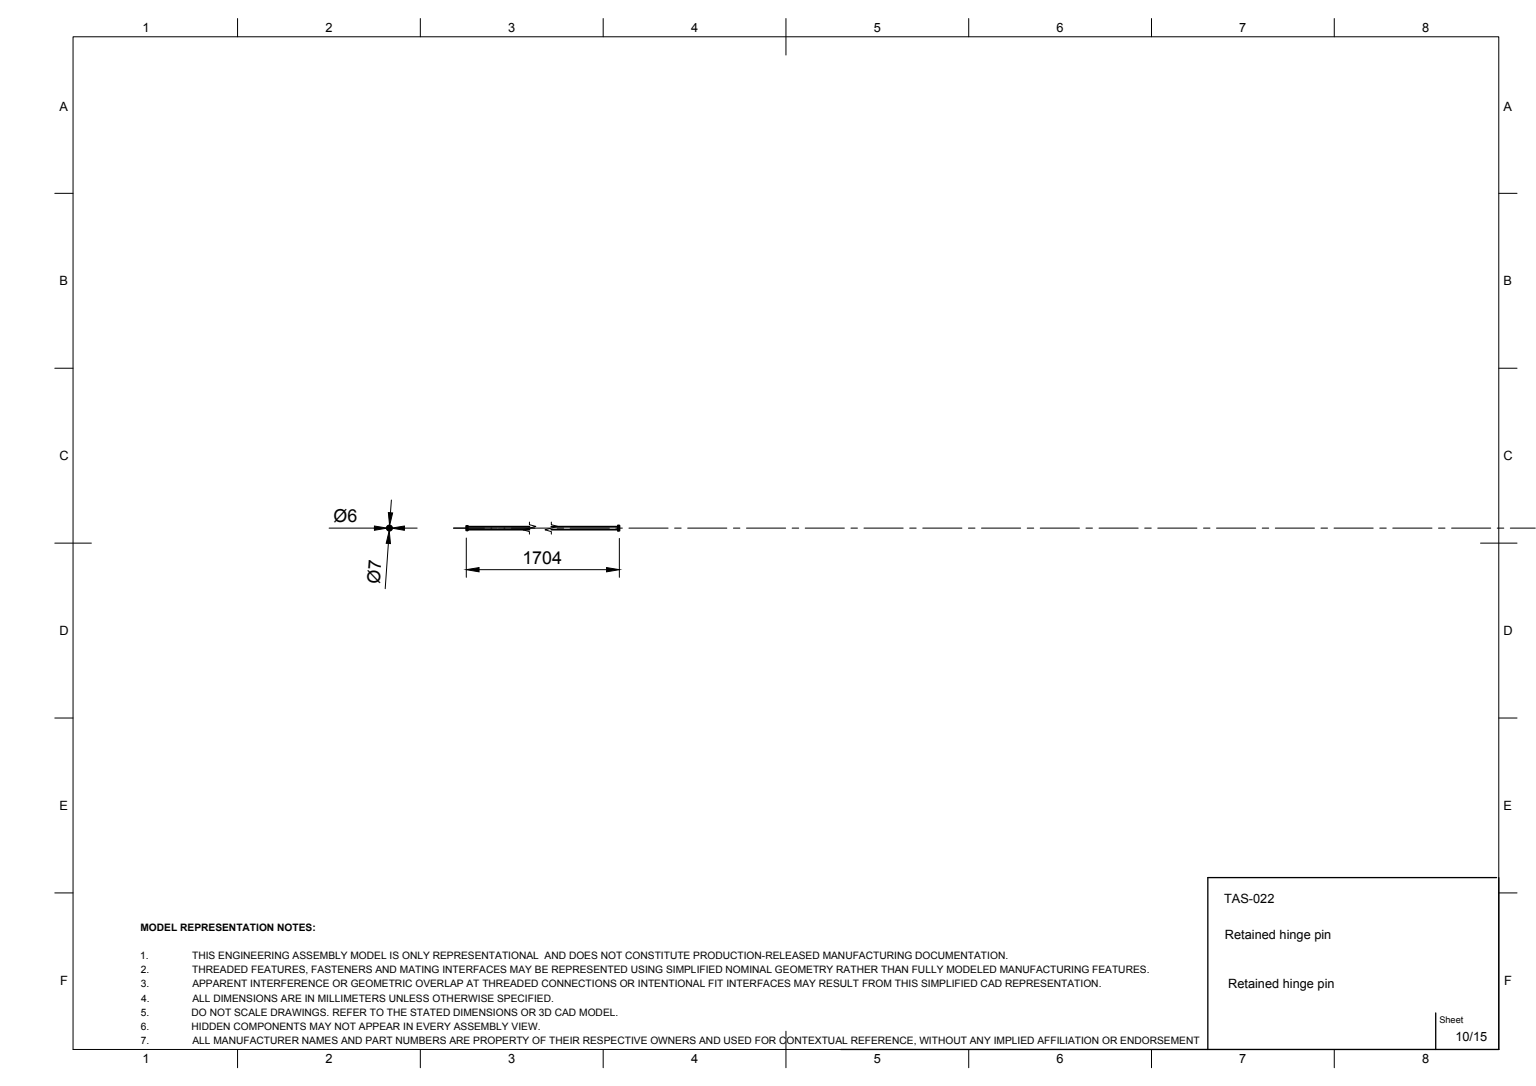
ISO-10303-21;
HEADER;
/* Generated by software containing ST-Developer
 * from STEP Tools, Inc. (www.steptools.com) 
 */

FILE_DESCRIPTION(
/* description */ (''),
/* implementation_level */ '2;1');

FILE_NAME(
/* name */ 'Retained hinge pin.step',
/* time_stamp */ '2026-11-15T21:02:08-08:00',
/* author */ (''),
/* organization */ (''),
/* preprocessor_version */ 'ST-DEVELOPER v20.2',
/* originating_system */ 'Autodesk Translation Framework v15.17.0.0',
/* authorisation */ '');

FILE_SCHEMA (('AUTOMOTIVE_DESIGN { 1 0 10303 214 3 1 1 }'));
ENDSEC;

DATA;
#10=MECHANICAL_DESIGN_GEOMETRIC_PRESENTATION_REPRESENTATION('',(#606),#31566);
#399=FACE_BOUND('',#972,.T.);
#400=FACE_BOUND('',#975,.T.);
#451=CIRCLE('',#5989,0.3);
#452=CIRCLE('',#5990,0.2);
#453=CIRCLE('',#5992,0.3);
#454=CIRCLE('',#5994,0.35);
#455=CIRCLE('',#5995,0.2);
#456=CIRCLE('',#5997,0.35);
#507=CYLINDRICAL_SURFACE('',#5991,0.3);
#508=CYLINDRICAL_SURFACE('',#5996,0.35);
#509=CYLINDRICAL_SURFACE('',#5999,0.2);
#576=SHAPE_REPRESENTATION_RELATIONSHIP('SRR','None',#31640,#591);
#591=ADVANCED_BREP_SHAPE_REPRESENTATION('',(#621),#31555);
#606=STYLED_ITEM('',(#31722),#621);
#621=MANIFOLD_SOLID_BREP('Body1',#5719);
#684=FACE_OUTER_BOUND('',#971,.T.);
#685=FACE_OUTER_BOUND('',#973,.T.);
#686=FACE_OUTER_BOUND('',#974,.T.);
#687=FACE_OUTER_BOUND('',#976,.T.);
#688=FACE_OUTER_BOUND('',#977,.T.);
#689=FACE_OUTER_BOUND('',#978,.T.);
#690=FACE_OUTER_BOUND('',#979,.T.);
#971=EDGE_LOOP('',(#3903));
#972=EDGE_LOOP('',(#3904));
#973=EDGE_LOOP('',(#3905,#3906,#3907,#3908));
#974=EDGE_LOOP('',(#3909));
#975=EDGE_LOOP('',(#3910));
#976=EDGE_LOOP('',(#3911,#3912,#3913,#3914));
#977=EDGE_LOOP('',(#3915));
#978=EDGE_LOOP('',(#3916,#3917,#3918,#3919));
#979=EDGE_LOOP('',(#3920));
#1310=LINE('',#7857,#1817);
#1311=LINE('',#7865,#1818);
#1312=LINE('',#7869,#1819);
#1817=VECTOR('',#6580,0.3);
#1818=VECTOR('',#6589,0.35);
#1819=VECTOR('',#6596,0.2);
#2312=VERTEX_POINT('',#7850);
#2313=VERTEX_POINT('',#7852);
#2314=VERTEX_POINT('',#7855);
#2315=VERTEX_POINT('',#7859);
#2316=VERTEX_POINT('',#7861);
#2317=VERTEX_POINT('',#7864);
#2947=EDGE_CURVE('',#2312,#2312,#451,.T.);
#2948=EDGE_CURVE('',#2313,#2313,#452,.T.);
#2949=EDGE_CURVE('',#2314,#2314,#453,.T.);
#2950=EDGE_CURVE('',#2314,#2312,#1310,.T.);
#2951=EDGE_CURVE('',#2315,#2315,#454,.T.);
#2952=EDGE_CURVE('',#2316,#2316,#455,.T.);
#2953=EDGE_CURVE('',#2315,#2317,#1311,.T.);
#2954=EDGE_CURVE('',#2317,#2317,#456,.T.);
#2955=EDGE_CURVE('',#2313,#2316,#1312,.T.);
#3903=ORIENTED_EDGE('',*,*,#2947,.F.);
#3904=ORIENTED_EDGE('',*,*,#2948,.F.);
#3905=ORIENTED_EDGE('',*,*,#2949,.F.);
#3906=ORIENTED_EDGE('',*,*,#2950,.T.);
#3907=ORIENTED_EDGE('',*,*,#2947,.T.);
#3908=ORIENTED_EDGE('',*,*,#2950,.F.);
#3909=ORIENTED_EDGE('',*,*,#2951,.T.);
#3910=ORIENTED_EDGE('',*,*,#2952,.F.);
#3911=ORIENTED_EDGE('',*,*,#2951,.F.);
#3912=ORIENTED_EDGE('',*,*,#2953,.T.);
#3913=ORIENTED_EDGE('',*,*,#2954,.T.);
#3914=ORIENTED_EDGE('',*,*,#2953,.F.);
#3915=ORIENTED_EDGE('',*,*,#2954,.F.);
#3916=ORIENTED_EDGE('',*,*,#2948,.T.);
#3917=ORIENTED_EDGE('',*,*,#2955,.T.);
#3918=ORIENTED_EDGE('',*,*,#2952,.T.);
#3919=ORIENTED_EDGE('',*,*,#2955,.F.);
#3920=ORIENTED_EDGE('',*,*,#2949,.T.);
#5298=PLANE('',#5988);
#5299=PLANE('',#5993);
#5300=PLANE('',#5998);
#5301=PLANE('',#6000);
#5498=ADVANCED_FACE('',(#684,#399),#5298,.F.);
#5499=ADVANCED_FACE('',(#685),#507,.T.);
#5500=ADVANCED_FACE('',(#686,#400),#5299,.T.);
#5501=ADVANCED_FACE('',(#687),#508,.T.);
#5502=ADVANCED_FACE('',(#688),#5300,.F.);
#5503=ADVANCED_FACE('',(#689),#509,.T.);
#5504=ADVANCED_FACE('',(#690),#5301,.T.);
#5719=CLOSED_SHELL('',(#5498,#5499,#5500,#5501,#5502,#5503,#5504));
#5987=AXIS2_PLACEMENT_3D('',#7848,#6568,#6569);
#5988=AXIS2_PLACEMENT_3D('',#7849,#6570,#6571);
#5989=AXIS2_PLACEMENT_3D('',#7851,#6572,#6573);
#5990=AXIS2_PLACEMENT_3D('',#7853,#6574,#6575);
#5991=AXIS2_PLACEMENT_3D('',#7854,#6576,#6577);
#5992=AXIS2_PLACEMENT_3D('',#7856,#6578,#6579);
#5993=AXIS2_PLACEMENT_3D('',#7858,#6581,#6582);
#5994=AXIS2_PLACEMENT_3D('',#7860,#6583,#6584);
#5995=AXIS2_PLACEMENT_3D('',#7862,#6585,#6586);
#5996=AXIS2_PLACEMENT_3D('',#7863,#6587,#6588);
#5997=AXIS2_PLACEMENT_3D('',#7866,#6590,#6591);
#5998=AXIS2_PLACEMENT_3D('',#7867,#6592,#6593);
#5999=AXIS2_PLACEMENT_3D('',#7868,#6594,#6595);
#6000=AXIS2_PLACEMENT_3D('',#7870,#6597,#6598);
#6568=DIRECTION('axis',(0.,0.,1.));
#6569=DIRECTION('refdir',(1.,0.,0.));
#6570=DIRECTION('center_axis',(0.,0.,1.));
#6571=DIRECTION('ref_axis',(1.,0.,0.));
#6572=DIRECTION('center_axis',(0.,0.,1.));
#6573=DIRECTION('ref_axis',(1.,0.,0.));
#6574=DIRECTION('center_axis',(0.,0.,-1.));
#6575=DIRECTION('ref_axis',(1.,0.,0.));
#6576=DIRECTION('center_axis',(0.,0.,1.));
#6577=DIRECTION('ref_axis',(1.,0.,0.));
#6578=DIRECTION('center_axis',(0.,0.,1.));
#6579=DIRECTION('ref_axis',(1.,0.,0.));
#6580=DIRECTION('',(0.,0.,-1.));
#6581=DIRECTION('center_axis',(0.,0.,1.));
#6582=DIRECTION('ref_axis',(1.,0.,0.));
#6583=DIRECTION('center_axis',(0.,0.,1.));
#6584=DIRECTION('ref_axis',(1.,0.,0.));
#6585=DIRECTION('center_axis',(0.,0.,1.));
#6586=DIRECTION('ref_axis',(1.,0.,0.));
#6587=DIRECTION('center_axis',(0.,0.,1.));
#6588=DIRECTION('ref_axis',(1.,0.,0.));
#6589=DIRECTION('',(0.,0.,-1.));
#6590=DIRECTION('center_axis',(0.,0.,1.));
#6591=DIRECTION('ref_axis',(1.,0.,0.));
#6592=DIRECTION('center_axis',(0.,0.,1.));
#6593=DIRECTION('ref_axis',(1.,0.,0.));
#6594=DIRECTION('center_axis',(0.,0.,1.));
#6595=DIRECTION('ref_axis',(1.,0.,0.));
#6596=DIRECTION('',(0.,0.,-1.));
#6597=DIRECTION('center_axis',(0.,0.,1.));
#6598=DIRECTION('ref_axis',(1.,0.,0.));
#7848=CARTESIAN_POINT('',(0.,0.,0.));
#7849=CARTESIAN_POINT('Origin',(0.,0.,170.));
#7850=CARTESIAN_POINT('',(-0.3,-3.67394039744206E-17,170.));
#7851=CARTESIAN_POINT('Origin',(0.,0.,170.));
#7852=CARTESIAN_POINT('',(-0.2,2.44929359829471E-17,170.));
#7853=CARTESIAN_POINT('Origin',(0.,0.,170.));
#7854=CARTESIAN_POINT('Origin',(0.,0.,170.));
#7855=CARTESIAN_POINT('',(-0.3,-3.67394039744206E-17,170.2));
#7856=CARTESIAN_POINT('Origin',(0.,0.,170.2));
#7857=CARTESIAN_POINT('',(-0.3,-3.67394039744206E-17,170.));
#7858=CARTESIAN_POINT('Origin',(0.,0.,0.));
#7859=CARTESIAN_POINT('',(-0.35,-4.28626379701574E-17,0.));
#7860=CARTESIAN_POINT('Origin',(0.,0.,0.));
#7861=CARTESIAN_POINT('',(-0.2,-2.44929359829471E-17,0.));
#7862=CARTESIAN_POINT('Origin',(0.,0.,0.));
#7863=CARTESIAN_POINT('Origin',(0.,0.,-0.2));
#7864=CARTESIAN_POINT('',(-0.35,-4.28626379701574E-17,-0.2));
#7865=CARTESIAN_POINT('',(-0.35,-4.28626379701574E-17,-0.2));
#7866=CARTESIAN_POINT('Origin',(0.,0.,-0.2));
#7867=CARTESIAN_POINT('Origin',(0.,0.,-0.2));
#7868=CARTESIAN_POINT('Origin',(0.,0.,0.));
#7869=CARTESIAN_POINT('',(-0.2,-2.44929359829471E-17,0.));
#7870=CARTESIAN_POINT('Origin',(0.,0.,170.2));
#31538=UNCERTAINTY_MEASURE_WITH_UNIT(LENGTH_MEASURE(0.001),#31567,
'DISTANCE_ACCURACY_VALUE',
'Maximum model space distance between geometric entities at asserted c
onnectivities');
#31549=UNCERTAINTY_MEASURE_WITH_UNIT(LENGTH_MEASURE(0.001),#31567,
'DISTANCE_ACCURACY_VALUE',
'Maximum model space distance between geometric entities at asserted c
onnectivities');
#31555=(
GEOMETRIC_REPRESENTATION_CONTEXT(3)
GLOBAL_UNCERTAINTY_ASSIGNED_CONTEXT((#31538))
GLOBAL_UNIT_ASSIGNED_CONTEXT((#31567,#31569,#31570))
REPRESENTATION_CONTEXT('','3D')
);
#31566=(
GEOMETRIC_REPRESENTATION_CONTEXT(3)
GLOBAL_UNCERTAINTY_ASSIGNED_CONTEXT((#31549))
GLOBAL_UNIT_ASSIGNED_CONTEXT((#31567,#31569,#31570))
REPRESENTATION_CONTEXT('','3D')
);
#31567=(
LENGTH_UNIT()
NAMED_UNIT(*)
SI_UNIT(.CENTI.,.METRE.)
);
#31569=(
NAMED_UNIT(*)
PLANE_ANGLE_UNIT()
SI_UNIT($,.RADIAN.)
);
#31570=(
NAMED_UNIT(*)
SI_UNIT($,.STERADIAN.)
SOLID_ANGLE_UNIT()
);
#31576=SHAPE_DEFINITION_REPRESENTATION(#31592,#31640);
#31592=PRODUCT_DEFINITION_SHAPE('',$,#31657);
#31640=SHAPE_REPRESENTATION('',(#5987),#31555);
#31651=PRODUCT_DEFINITION_CONTEXT('part definition',#31701,'design');
#31657=PRODUCT_DEFINITION('Retained hinge pin','Retained hinge pin',#31673,
#31651);
#31673=PRODUCT_DEFINITION_FORMATION('',$,#31708);
#31701=APPLICATION_CONTEXT(
'Core Data for Automotive Mechanical Design Process');
#31702=PRODUCT_CONTEXT('part definition',#31701,'mechanical');
#31708=PRODUCT('Retained hinge pin','Retained hinge pin',$,(#31702));
#31722=PRESENTATION_STYLE_ASSIGNMENT((#31729));
#31729=SURFACE_STYLE_USAGE(.BOTH.,#31736);
#31736=SURFACE_SIDE_STYLE('',(#31743));
#31743=SURFACE_STYLE_FILL_AREA(#31750);
#31750=FILL_AREA_STYLE('Opaque(75,81,92)',(#31757));
#31757=FILL_AREA_STYLE_COLOUR('Opaque(75,81,92)',#31764);
#31764=COLOUR_RGB('Opaque(75,81,92)',0.294117647058824,0.317647058823529,
0.36078431372549);
ENDSEC;
END-ISO-10303-21;
